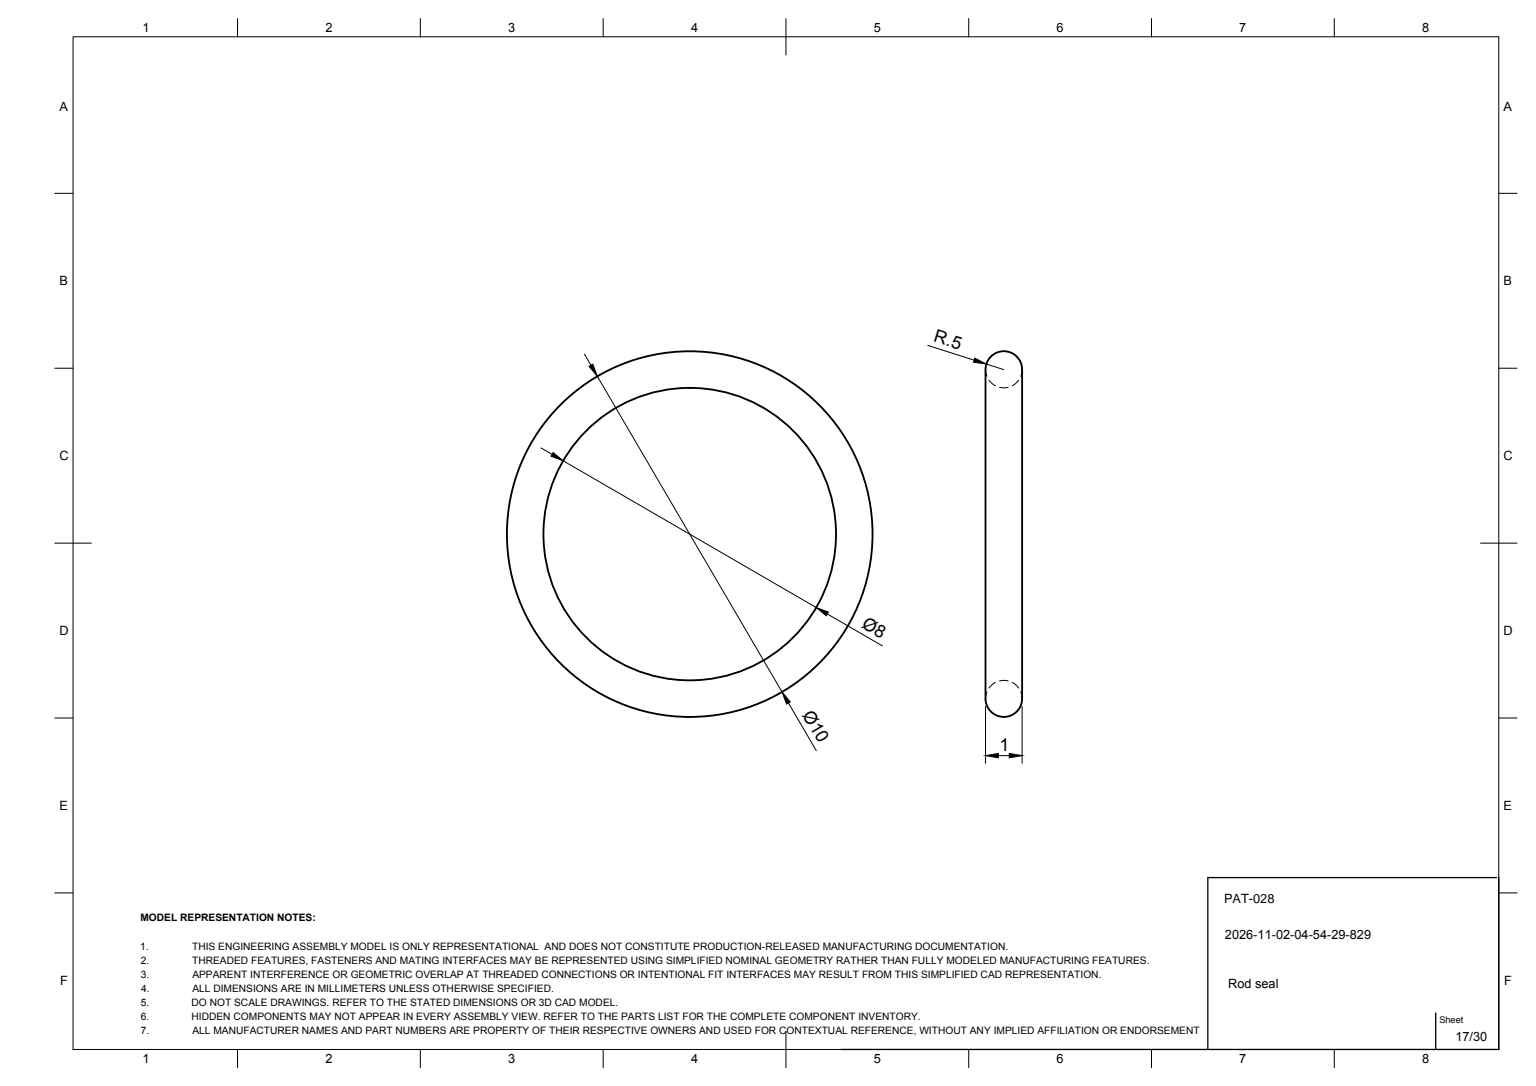
ISO-10303-21;
HEADER;
/* Generated by software containing ST-Developer
 * from STEP Tools, Inc. (www.steptools.com) 
 */

FILE_DESCRIPTION(
/* description */ ('Cylinder foot and clevis mount kit'),
/* implementation_level */ '2;1');

FILE_NAME(
/* name */ 'Rod seal.step',
/* time_stamp */ '2026-10-27T20:10:43-07:00',
/* author */ (''),
/* organization */ (''),
/* preprocessor_version */ 'ST-DEVELOPER v20.2',
/* originating_system */ 'Autodesk Translation Framework v15.17.0.0',
/* authorisation */ '');

FILE_SCHEMA (('AUTOMOTIVE_DESIGN { 1 0 10303 214 3 1 1 }'));
ENDSEC;

DATA;
#10=MECHANICAL_DESIGN_GEOMETRIC_PRESENTATION_REPRESENTATION('',(#353),#9102);
#32=TOROIDAL_SURFACE('',#5660,0.45,0.05);
#297=SHAPE_REPRESENTATION_RELATIONSHIP('SRR','None',#9245,#325);
#325=ADVANCED_BREP_SHAPE_REPRESENTATION('',(#380),#9088);
#353=STYLED_ITEM('',(#9467),#380);
#380=MANIFOLD_SOLID_BREP('Body1',#4940);
#903=FACE_OUTER_BOUND('',#1287,.T.);
#1287=EDGE_LOOP('',(#4133,#4134,#4135,#4136));
#2262=CIRCLE('',#5661,0.05);
#2263=CIRCLE('',#5662,0.4);
#2587=VERTEX_POINT('',#8394);
#3121=EDGE_CURVE('',#2587,#2587,#2262,.T.);
#3122=EDGE_CURVE('',#2587,#2587,#2263,.T.);
#4133=ORIENTED_EDGE('',*,*,#3121,.F.);
#4134=ORIENTED_EDGE('',*,*,#3122,.T.);
#4135=ORIENTED_EDGE('',*,*,#3121,.T.);
#4136=ORIENTED_EDGE('',*,*,#3122,.F.);
#4826=ADVANCED_FACE('',(#903),#32,.T.);
#4940=CLOSED_SHELL('',(#4826));
#5659=AXIS2_PLACEMENT_3D('',#8392,#6924,#6925);
#5660=AXIS2_PLACEMENT_3D('',#8393,#6926,#6927);
#5661=AXIS2_PLACEMENT_3D('',#8395,#6928,#6929);
#5662=AXIS2_PLACEMENT_3D('',#8396,#6930,#6931);
#6924=DIRECTION('axis',(0.,0.,1.));
#6925=DIRECTION('refdir',(1.,0.,0.));
#6926=DIRECTION('center_axis',(0.,-1.,0.));
#6927=DIRECTION('ref_axis',(0.,0.,-1.));
#6928=DIRECTION('center_axis',(-1.,0.,-1.22464679914735E-16));
#6929=DIRECTION('ref_axis',(-1.22464679914735E-16,0.,1.));
#6930=DIRECTION('center_axis',(0.,1.,0.));
#6931=DIRECTION('ref_axis',(0.,0.,-1.));
#8392=CARTESIAN_POINT('',(0.,0.,0.));
#8393=CARTESIAN_POINT('Origin',(0.,0.2,4.5));
#8394=CARTESIAN_POINT('',(-4.89858719658941E-17,0.2,4.9));
#8395=CARTESIAN_POINT('Origin',(-5.51091059616309E-17,0.2,4.95));
#8396=CARTESIAN_POINT('Origin',(0.,0.2,4.5));
#9055=UNCERTAINTY_MEASURE_WITH_UNIT(LENGTH_MEASURE(0.001),#9103,
'DISTANCE_ACCURACY_VALUE',
'Maximum model space distance between geometric entities at asserted c
onnectivities');
#9069=UNCERTAINTY_MEASURE_WITH_UNIT(LENGTH_MEASURE(0.001),#9103,
'DISTANCE_ACCURACY_VALUE',
'Maximum model space distance between geometric entities at asserted c
onnectivities');
#9088=(
GEOMETRIC_REPRESENTATION_CONTEXT(3)
GLOBAL_UNCERTAINTY_ASSIGNED_CONTEXT((#9055))
GLOBAL_UNIT_ASSIGNED_CONTEXT((#9103,#9105,#9106))
REPRESENTATION_CONTEXT('','3D')
);
#9102=(
GEOMETRIC_REPRESENTATION_CONTEXT(3)
GLOBAL_UNCERTAINTY_ASSIGNED_CONTEXT((#9069))
GLOBAL_UNIT_ASSIGNED_CONTEXT((#9103,#9105,#9106))
REPRESENTATION_CONTEXT('','3D')
);
#9103=(
LENGTH_UNIT()
NAMED_UNIT(*)
SI_UNIT(.CENTI.,.METRE.)
);
#9105=(
NAMED_UNIT(*)
PLANE_ANGLE_UNIT()
SI_UNIT($,.RADIAN.)
);
#9106=(
NAMED_UNIT(*)
SI_UNIT($,.STERADIAN.)
SOLID_ANGLE_UNIT()
);
#9125=SHAPE_DEFINITION_REPRESENTATION(#9159,#9245);
#9159=PRODUCT_DEFINITION_SHAPE('',$,#9278);
#9245=SHAPE_REPRESENTATION('',(#5659),#9088);
#9259=PRODUCT_DEFINITION_CONTEXT('part definition',#9357,'design');
#9278=PRODUCT_DEFINITION('Rod seal','Rod seal',#9310,#9259);
#9310=PRODUCT_DEFINITION_FORMATION('',$,#9377);
#9357=APPLICATION_CONTEXT(
'Core Data for Automotive Mechanical Design Process');
#9358=PRODUCT_CONTEXT('part definition',#9357,'mechanical');
#9377=PRODUCT('Rod seal','Rod seal','Rod seal',(#9358));
#9461=COLOUR_RGB('Black',0.12,0.14,0.17);
#9462=FILL_AREA_STYLE_COLOUR('',#9461);
#9463=FILL_AREA_STYLE('',(#9462));
#9464=SURFACE_STYLE_FILL_AREA(#9463);
#9465=SURFACE_SIDE_STYLE('',(#9464));
#9466=SURFACE_STYLE_USAGE(.BOTH.,#9465);
#9467=PRESENTATION_STYLE_ASSIGNMENT((#9466));
ENDSEC;
END-ISO-10303-21;
